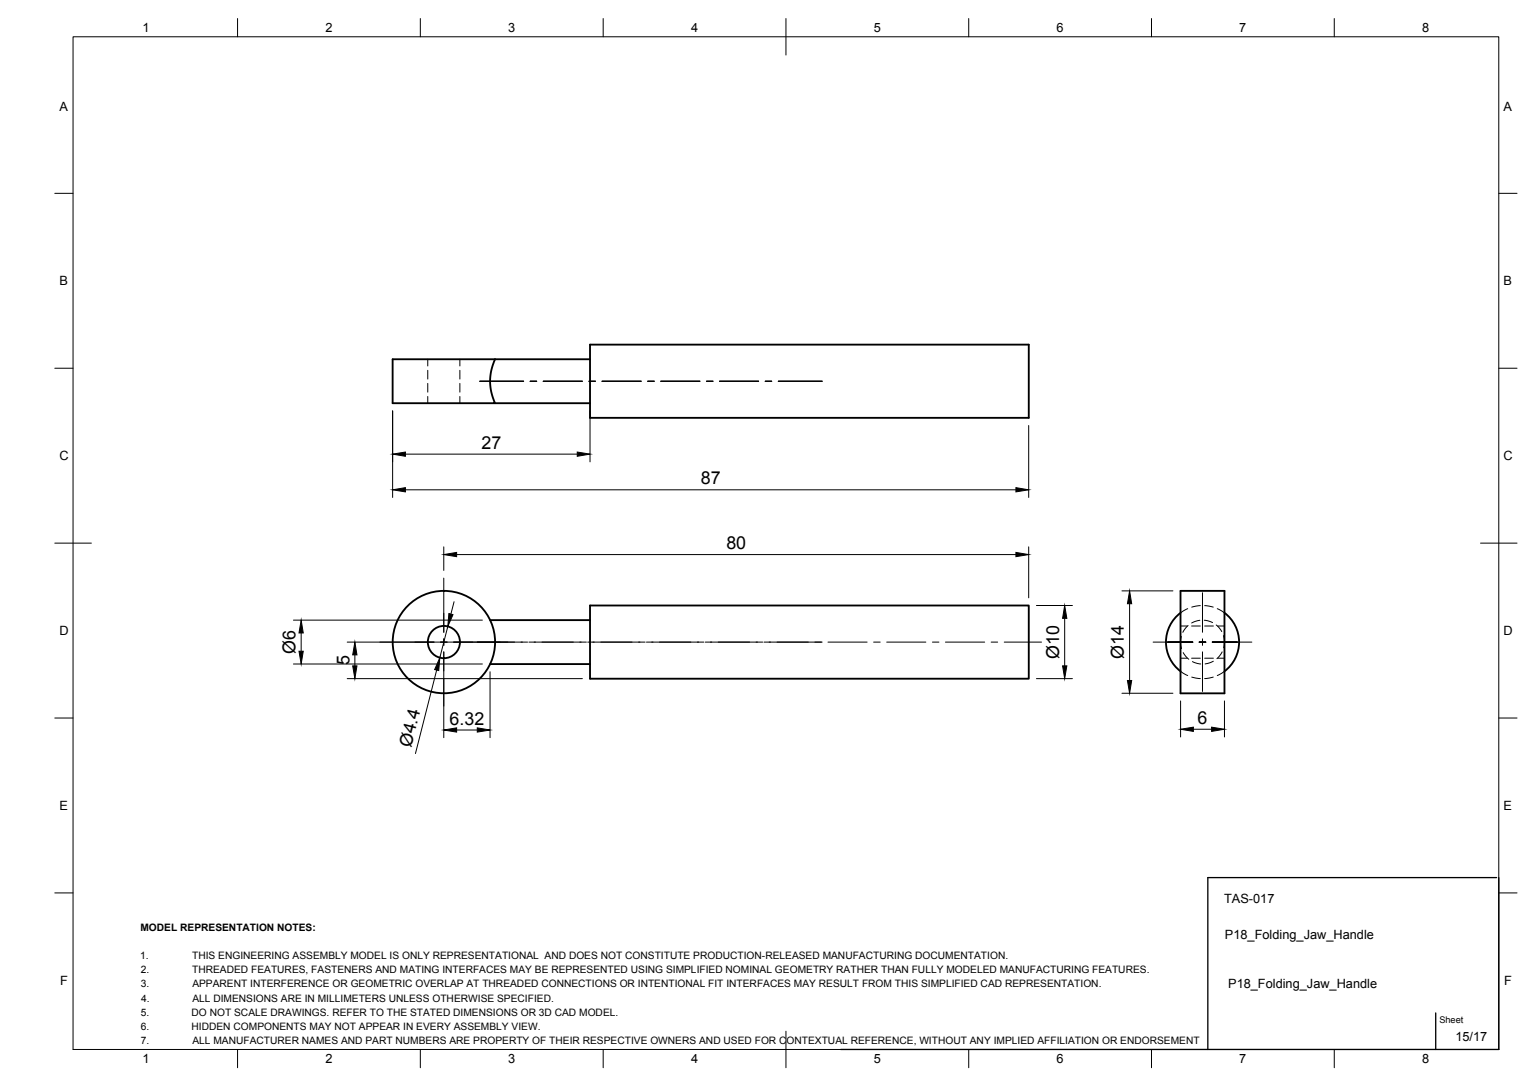
ISO-10303-21;
HEADER;
/* Generated by software containing ST-Developer
 * from STEP Tools, Inc. (www.steptools.com) 
 */

FILE_DESCRIPTION(
/* description */ ('STEP AP203'),
/* implementation_level */ '2;1');

FILE_NAME(
/* name */ 'P18_Folding_Jaw_Handle.step',
/* time_stamp */ '2026-11-15T15:04:01-08:00',
/* author */ (''),
/* organization */ (''),
/* preprocessor_version */ 'ST-DEVELOPER v20.2',
/* originating_system */ 'Autodesk Translation Framework v15.17.0.0',
/* authorisation */ '');

FILE_SCHEMA (('AUTOMOTIVE_DESIGN { 1 0 10303 214 3 1 1 }'));
ENDSEC;

DATA;
#10=MECHANICAL_DESIGN_GEOMETRIC_PRESENTATION_REPRESENTATION('',(#294),#16598);
#193=B_SPLINE_CURVE_WITH_KNOTS('',3,(#14963,#14964,#14965,#14966,#14967,
#14968,#14969,#14970,#14971,#14972,#14973,#14974,#14975,#14976,#14977,#14978,
#14979,#14980),.UNSPECIFIED.,.F.,.F.,(4,2,2,2,2,2,2,2,4),(0.458554765704034,
0.573115036583473,0.687675307462911,0.80239241943549,0.917109531408068,
1.03182664338065,1.14654375535323,1.26110402623266,1.3756642971121),
 .UNSPECIFIED.);
#194=B_SPLINE_CURVE_WITH_KNOTS('',3,(#14982,#14983,#14984,#14985,#14986,
#14987,#14988,#14989,#14990,#14991,#14992,#14993,#14994,#14995,#14996,#14997,
#14998,#14999,#15000),.UNSPECIFIED.,.F.,.F.,(4,2,2,2,3,2,2,2,4),(-0.458554765704034,
-0.343994494824596,-0.229434223945157,-0.114717111972579,0.,0.114717111972579,
0.229434223945157,0.343994494824596,0.458554765704034),.UNSPECIFIED.);
#216=SHAPE_REPRESENTATION_RELATIONSHIP('SRR','None',#16710,#240);
#240=ADVANCED_BREP_SHAPE_REPRESENTATION('',(#264),#16586);
#264=MANIFOLD_SOLID_BREP('Body1',#9799);
#294=STYLED_ITEM('',(#16832),#264);
#359=FACE_BOUND('',#1759,.T.);
#360=FACE_BOUND('',#1762,.T.);
#361=FACE_BOUND('',#1764,.T.);
#627=PLANE('',#10436);
#628=PLANE('',#10437);
#629=PLANE('',#10438);
#630=PLANE('',#10439);
#1150=FACE_OUTER_BOUND('',#1754,.T.);
#1151=FACE_OUTER_BOUND('',#1755,.T.);
#1152=FACE_OUTER_BOUND('',#1756,.T.);
#1153=FACE_OUTER_BOUND('',#1757,.T.);
#1154=FACE_OUTER_BOUND('',#1758,.T.);
#1155=FACE_OUTER_BOUND('',#1760,.T.);
#1156=FACE_OUTER_BOUND('',#1761,.T.);
#1157=FACE_OUTER_BOUND('',#1763,.T.);
#1754=EDGE_LOOP('',(#7737,#7738,#7739,#7740));
#1755=EDGE_LOOP('',(#7741,#7742,#7743,#7744));
#1756=EDGE_LOOP('',(#7745,#7746,#7747,#7748));
#1757=EDGE_LOOP('',(#7749,#7750,#7751,#7752,#7753));
#1758=EDGE_LOOP('',(#7754));
#1759=EDGE_LOOP('',(#7755));
#1760=EDGE_LOOP('',(#7756));
#1761=EDGE_LOOP('',(#7757));
#1762=EDGE_LOOP('',(#7758));
#1763=EDGE_LOOP('',(#7759));
#1764=EDGE_LOOP('',(#7760));
#2606=LINE('',#14957,#3654);
#2607=LINE('',#15005,#3655);
#2608=LINE('',#15010,#3656);
#3654=VECTOR('',#12100,2.19999999999999);
#3655=VECTOR('',#12113,5.);
#3656=VECTOR('',#12120,3.);
#4319=CIRCLE('',#10426,2.19999999999999);
#4320=CIRCLE('',#10427,2.19999999999999);
#4321=CIRCLE('',#10429,7.00000000000001);
#4322=CIRCLE('',#10430,7.00000000000001);
#4323=CIRCLE('',#10432,5.);
#4324=CIRCLE('',#10433,5.);
#4325=CIRCLE('',#10435,3.);
#4835=VERTEX_POINT('',#14954);
#4836=VERTEX_POINT('',#14956);
#4837=VERTEX_POINT('',#14960);
#4838=VERTEX_POINT('',#14962);
#4839=VERTEX_POINT('',#15002);
#4840=VERTEX_POINT('',#15004);
#4841=VERTEX_POINT('',#15008);
#5881=EDGE_CURVE('',#4835,#4835,#4319,.T.);
#5882=EDGE_CURVE('',#4835,#4836,#2606,.T.);
#5883=EDGE_CURVE('',#4836,#4836,#4320,.T.);
#5884=EDGE_CURVE('',#4837,#4837,#4321,.T.);
#5885=EDGE_CURVE('',#4837,#4838,#193,.T.);
#5886=EDGE_CURVE('',#4838,#4838,#4322,.T.);
#5887=EDGE_CURVE('',#4838,#4837,#194,.T.);
#5888=EDGE_CURVE('',#4839,#4839,#4323,.T.);
#5889=EDGE_CURVE('',#4839,#4840,#2607,.T.);
#5890=EDGE_CURVE('',#4840,#4840,#4324,.T.);
#5891=EDGE_CURVE('',#4841,#4841,#4325,.T.);
#5892=EDGE_CURVE('',#4841,#4837,#2608,.T.);
#7737=ORIENTED_EDGE('',*,*,#5881,.F.);
#7738=ORIENTED_EDGE('',*,*,#5882,.T.);
#7739=ORIENTED_EDGE('',*,*,#5883,.T.);
#7740=ORIENTED_EDGE('',*,*,#5882,.F.);
#7741=ORIENTED_EDGE('',*,*,#5884,.F.);
#7742=ORIENTED_EDGE('',*,*,#5885,.T.);
#7743=ORIENTED_EDGE('',*,*,#5886,.T.);
#7744=ORIENTED_EDGE('',*,*,#5887,.T.);
#7745=ORIENTED_EDGE('',*,*,#5888,.T.);
#7746=ORIENTED_EDGE('',*,*,#5889,.T.);
#7747=ORIENTED_EDGE('',*,*,#5890,.F.);
#7748=ORIENTED_EDGE('',*,*,#5889,.F.);
#7749=ORIENTED_EDGE('',*,*,#5891,.T.);
#7750=ORIENTED_EDGE('',*,*,#5892,.T.);
#7751=ORIENTED_EDGE('',*,*,#5887,.F.);
#7752=ORIENTED_EDGE('',*,*,#5885,.F.);
#7753=ORIENTED_EDGE('',*,*,#5892,.F.);
#7754=ORIENTED_EDGE('',*,*,#5890,.T.);
#7755=ORIENTED_EDGE('',*,*,#5891,.F.);
#7756=ORIENTED_EDGE('',*,*,#5888,.F.);
#7757=ORIENTED_EDGE('',*,*,#5884,.T.);
#7758=ORIENTED_EDGE('',*,*,#5881,.T.);
#7759=ORIENTED_EDGE('',*,*,#5886,.F.);
#7760=ORIENTED_EDGE('',*,*,#5883,.F.);
#9210=CYLINDRICAL_SURFACE('',#10425,2.19999999999999);
#9211=CYLINDRICAL_SURFACE('',#10428,7.00000000000001);
#9212=CYLINDRICAL_SURFACE('',#10431,5.);
#9213=CYLINDRICAL_SURFACE('',#10434,3.);
#9475=ADVANCED_FACE('',(#1150),#9210,.F.);
#9476=ADVANCED_FACE('',(#1151),#9211,.T.);
#9477=ADVANCED_FACE('',(#1152),#9212,.T.);
#9478=ADVANCED_FACE('',(#1153),#9213,.T.);
#9479=ADVANCED_FACE('',(#1154,#359),#627,.T.);
#9480=ADVANCED_FACE('',(#1155),#628,.F.);
#9481=ADVANCED_FACE('',(#1156,#360),#629,.T.);
#9482=ADVANCED_FACE('',(#1157,#361),#630,.F.);
#9799=CLOSED_SHELL('',(#9475,#9476,#9477,#9478,#9479,#9480,#9481,#9482));
#10424=AXIS2_PLACEMENT_3D('',#14952,#12094,#12095);
#10425=AXIS2_PLACEMENT_3D('',#14953,#12096,#12097);
#10426=AXIS2_PLACEMENT_3D('',#14955,#12098,#12099);
#10427=AXIS2_PLACEMENT_3D('',#14958,#12101,#12102);
#10428=AXIS2_PLACEMENT_3D('',#14959,#12103,#12104);
#10429=AXIS2_PLACEMENT_3D('',#14961,#12105,#12106);
#10430=AXIS2_PLACEMENT_3D('',#14981,#12107,#12108);
#10431=AXIS2_PLACEMENT_3D('',#15001,#12109,#12110);
#10432=AXIS2_PLACEMENT_3D('',#15003,#12111,#12112);
#10433=AXIS2_PLACEMENT_3D('',#15006,#12114,#12115);
#10434=AXIS2_PLACEMENT_3D('',#15007,#12116,#12117);
#10435=AXIS2_PLACEMENT_3D('',#15009,#12118,#12119);
#10436=AXIS2_PLACEMENT_3D('',#15011,#12121,#12122);
#10437=AXIS2_PLACEMENT_3D('',#15012,#12123,#12124);
#10438=AXIS2_PLACEMENT_3D('',#15013,#12125,#12126);
#10439=AXIS2_PLACEMENT_3D('',#15014,#12127,#12128);
#12094=DIRECTION('axis',(0.,0.,1.));
#12095=DIRECTION('refdir',(1.,0.,0.));
#12096=DIRECTION('center_axis',(-1.,0.,0.));
#12097=DIRECTION('ref_axis',(0.,0.,1.));
#12098=DIRECTION('center_axis',(-1.,0.,0.));
#12099=DIRECTION('ref_axis',(0.,0.,-1.));
#12100=DIRECTION('',(-1.,0.,0.));
#12101=DIRECTION('center_axis',(-1.,0.,0.));
#12102=DIRECTION('ref_axis',(0.,0.,-1.));
#12103=DIRECTION('center_axis',(-1.,0.,0.));
#12104=DIRECTION('ref_axis',(0.,0.,1.));
#12105=DIRECTION('center_axis',(1.,0.,0.));
#12106=DIRECTION('ref_axis',(0.,0.,-1.));
#12107=DIRECTION('center_axis',(1.,0.,0.));
#12108=DIRECTION('ref_axis',(0.,0.,-1.));
#12109=DIRECTION('center_axis',(0.,0.,-1.));
#12110=DIRECTION('ref_axis',(-1.,0.,0.));
#12111=DIRECTION('center_axis',(0.,0.,1.));
#12112=DIRECTION('ref_axis',(1.,0.,0.));
#12113=DIRECTION('',(0.,0.,1.));
#12114=DIRECTION('center_axis',(0.,0.,1.));
#12115=DIRECTION('ref_axis',(1.,0.,0.));
#12116=DIRECTION('center_axis',(0.,0.,-1.));
#12117=DIRECTION('ref_axis',(-1.,0.,0.));
#12118=DIRECTION('center_axis',(0.,0.,1.));
#12119=DIRECTION('ref_axis',(1.,0.,0.));
#12120=DIRECTION('',(0.,0.,1.));
#12121=DIRECTION('center_axis',(0.,0.,1.));
#12122=DIRECTION('ref_axis',(1.,0.,0.));
#12123=DIRECTION('center_axis',(0.,0.,1.));
#12124=DIRECTION('ref_axis',(1.,0.,0.));
#12125=DIRECTION('center_axis',(1.,0.,0.));
#12126=DIRECTION('ref_axis',(0.,0.,-1.));
#12127=DIRECTION('center_axis',(1.,0.,0.));
#12128=DIRECTION('ref_axis',(0.,0.,-1.));
#14952=CARTESIAN_POINT('',(0.,0.,0.));
#14953=CARTESIAN_POINT('Origin',(4.,0.,80.));
#14954=CARTESIAN_POINT('',(3.,-2.69422295812417E-16,77.8));
#14955=CARTESIAN_POINT('Origin',(3.,0.,80.));
#14956=CARTESIAN_POINT('',(-3.,-2.69422295812417E-16,77.8));
#14957=CARTESIAN_POINT('',(4.,-2.69422295812417E-16,77.8));
#14958=CARTESIAN_POINT('Origin',(-3.,0.,80.));
#14959=CARTESIAN_POINT('Origin',(3.,0.,80.));
#14960=CARTESIAN_POINT('',(3.,-6.21185679917027E-21,73.));
#14961=CARTESIAN_POINT('Origin',(3.,0.,80.));
#14962=CARTESIAN_POINT('',(-3.,0.,73.));
#14963=CARTESIAN_POINT('Ctrl Pts',(3.,4.5102810375397E-16,73.));
#14964=CARTESIAN_POINT('Ctrl Pts',(3.,0.381867569598129,73.));
#14965=CARTESIAN_POINT('Ctrl Pts',(2.92268305871952,0.785938626528129,73.0342116500025));
#14966=CARTESIAN_POINT('Ctrl Pts',(2.61493784812886,1.52377016291608,73.1576296998384));
#14967=CARTESIAN_POINT('Ctrl Pts',(2.38476353394969,1.8578771531696,73.2453932009422));
#14968=CARTESIAN_POINT('Ctrl Pts',(1.85751648085586,2.38512420626343,73.4130574284979));
#14969=CARTESIAN_POINT('Ctrl Pts',(1.52354231756781,2.61502716928633,73.5046430803547));
#14970=CARTESIAN_POINT('Ctrl Pts',(0.786243067181792,2.92256178949426,73.6370868756761));
#14971=CARTESIAN_POINT('Ctrl Pts',(0.382390373241929,3.,73.6754446796632));
#14972=CARTESIAN_POINT('Ctrl Pts',(-0.382390373241929,3.,73.6754446796632));
#14973=CARTESIAN_POINT('Ctrl Pts',(-0.786243067181794,2.92256178949426,
73.6370868756761));
#14974=CARTESIAN_POINT('Ctrl Pts',(-1.52354231756781,2.61502716928633,73.5046430803547));
#14975=CARTESIAN_POINT('Ctrl Pts',(-1.85751648085586,2.38512420626343,73.4130574284979));
#14976=CARTESIAN_POINT('Ctrl Pts',(-2.38476353394969,1.8578771531696,73.2453932009422));
#14977=CARTESIAN_POINT('Ctrl Pts',(-2.61493784812886,1.52377016291608,73.1576296998384));
#14978=CARTESIAN_POINT('Ctrl Pts',(-2.92268305871952,0.785938626528129,
73.0342116500025));
#14979=CARTESIAN_POINT('Ctrl Pts',(-3.,0.381867569598128,73.));
#14980=CARTESIAN_POINT('Ctrl Pts',(-3.,0.,73.));
#14981=CARTESIAN_POINT('Origin',(-3.,0.,80.));
#14982=CARTESIAN_POINT('Ctrl Pts',(-3.,6.59194920871187E-16,73.));
#14983=CARTESIAN_POINT('Ctrl Pts',(-3.,-0.381867569598127,73.));
#14984=CARTESIAN_POINT('Ctrl Pts',(-2.92268305871952,-0.785938626528129,
73.0342116500025));
#14985=CARTESIAN_POINT('Ctrl Pts',(-2.61493784812886,-1.52377016291608,
73.1576296998384));
#14986=CARTESIAN_POINT('Ctrl Pts',(-2.38476353394969,-1.8578771531696,73.2453932009422));
#14987=CARTESIAN_POINT('Ctrl Pts',(-1.85751648085586,-2.38512420626343,
73.4130574284979));
#14988=CARTESIAN_POINT('Ctrl Pts',(-1.52354231756781,-2.61502716928633,
73.5046430803547));
#14989=CARTESIAN_POINT('Ctrl Pts',(-0.786243067181791,-2.92256178949426,
73.6370868756761));
#14990=CARTESIAN_POINT('Ctrl Pts',(-0.382390373241929,-3.,73.6754446796632));
#14991=CARTESIAN_POINT('Ctrl Pts',(0.,-3.,73.6754446796632));
#14992=CARTESIAN_POINT('Ctrl Pts',(0.382390373241929,-3.,73.6754446796632));
#14993=CARTESIAN_POINT('Ctrl Pts',(0.786243067181791,-2.92256178949426,
73.6370868756761));
#14994=CARTESIAN_POINT('Ctrl Pts',(1.52354231756781,-2.61502716928633,73.5046430803547));
#14995=CARTESIAN_POINT('Ctrl Pts',(1.85751648085586,-2.38512420626343,73.4130574284979));
#14996=CARTESIAN_POINT('Ctrl Pts',(2.38476353394969,-1.8578771531696,73.2453932009422));
#14997=CARTESIAN_POINT('Ctrl Pts',(2.61493784812886,-1.52377016291608,73.1576296998384));
#14998=CARTESIAN_POINT('Ctrl Pts',(2.92268305871952,-0.785938626528129,
73.0342116500025));
#14999=CARTESIAN_POINT('Ctrl Pts',(3.,-0.381867569598129,73.));
#15000=CARTESIAN_POINT('Ctrl Pts',(3.,-4.85722573273506E-16,73.));
#15001=CARTESIAN_POINT('Origin',(0.,0.,60.));
#15002=CARTESIAN_POINT('',(5.,-6.12323399573677E-16,0.));
#15003=CARTESIAN_POINT('Origin',(0.,0.,0.));
#15004=CARTESIAN_POINT('',(5.,-6.12323399573677E-16,60.));
#15005=CARTESIAN_POINT('',(5.,-6.12323399573677E-16,60.));
#15006=CARTESIAN_POINT('Origin',(0.,0.,60.));
#15007=CARTESIAN_POINT('Origin',(0.,0.,80.));
#15008=CARTESIAN_POINT('',(3.,-3.67394039744206E-16,60.));
#15009=CARTESIAN_POINT('Origin',(0.,0.,60.));
#15010=CARTESIAN_POINT('',(3.,-3.67394039744206E-16,80.));
#15011=CARTESIAN_POINT('Origin',(0.,0.,60.));
#15012=CARTESIAN_POINT('Origin',(0.,0.,0.));
#15013=CARTESIAN_POINT('Origin',(3.,0.,80.));
#15014=CARTESIAN_POINT('Origin',(-3.,0.,80.));
#16560=UNCERTAINTY_MEASURE_WITH_UNIT(LENGTH_MEASURE(0.01),#16599,
'DISTANCE_ACCURACY_VALUE',
'Maximum model space distance between geometric entities at asserted c
onnectivities');
#16572=UNCERTAINTY_MEASURE_WITH_UNIT(LENGTH_MEASURE(0.01),#16599,
'DISTANCE_ACCURACY_VALUE',
'Maximum model space distance between geometric entities at asserted c
onnectivities');
#16586=(
GEOMETRIC_REPRESENTATION_CONTEXT(3)
GLOBAL_UNCERTAINTY_ASSIGNED_CONTEXT((#16560))
GLOBAL_UNIT_ASSIGNED_CONTEXT((#16599,#16601,#16602))
REPRESENTATION_CONTEXT('','3D')
);
#16598=(
GEOMETRIC_REPRESENTATION_CONTEXT(3)
GLOBAL_UNCERTAINTY_ASSIGNED_CONTEXT((#16572))
GLOBAL_UNIT_ASSIGNED_CONTEXT((#16599,#16601,#16602))
REPRESENTATION_CONTEXT('','3D')
);
#16599=(
LENGTH_UNIT()
NAMED_UNIT(*)
SI_UNIT(.MILLI.,.METRE.)
);
#16601=(
NAMED_UNIT(*)
PLANE_ANGLE_UNIT()
SI_UNIT($,.RADIAN.)
);
#16602=(
NAMED_UNIT(*)
SI_UNIT($,.STERADIAN.)
SOLID_ANGLE_UNIT()
);
#16616=SHAPE_DEFINITION_REPRESENTATION(#16641,#16710);
#16641=PRODUCT_DEFINITION_SHAPE('',$,#16736);
#16710=SHAPE_REPRESENTATION('',(#10424),#16586);
#16722=PRODUCT_DEFINITION_CONTEXT('part definition',#16799,'design');
#16736=PRODUCT_DEFINITION('P18_Folding_Jaw_Handle',
'P18_Folding_Jaw_Handle',#16761,#16722);
#16761=PRODUCT_DEFINITION_FORMATION('',$,#16814);
#16799=APPLICATION_CONTEXT(
'Core Data for Automotive Mechanical Design Process');
#16800=PRODUCT_CONTEXT('part definition',#16799,'mechanical');
#16814=PRODUCT('P18_Folding_Jaw_Handle','P18_Folding_Jaw_Handle',$,(#16800));
#16832=PRESENTATION_STYLE_ASSIGNMENT((#16841));
#16841=SURFACE_STYLE_USAGE(.BOTH.,#16850);
#16850=SURFACE_SIDE_STYLE('',(#16859));
#16859=SURFACE_STYLE_FILL_AREA(#16868);
#16868=FILL_AREA_STYLE('Sky Blue',(#16877));
#16877=FILL_AREA_STYLE_COLOUR('Sky Blue',#16886);
#16886=COLOUR_RGB('Sky Blue',0.529411764705882,0.807843137254902,0.92156862745098);
ENDSEC;
END-ISO-10303-21;
